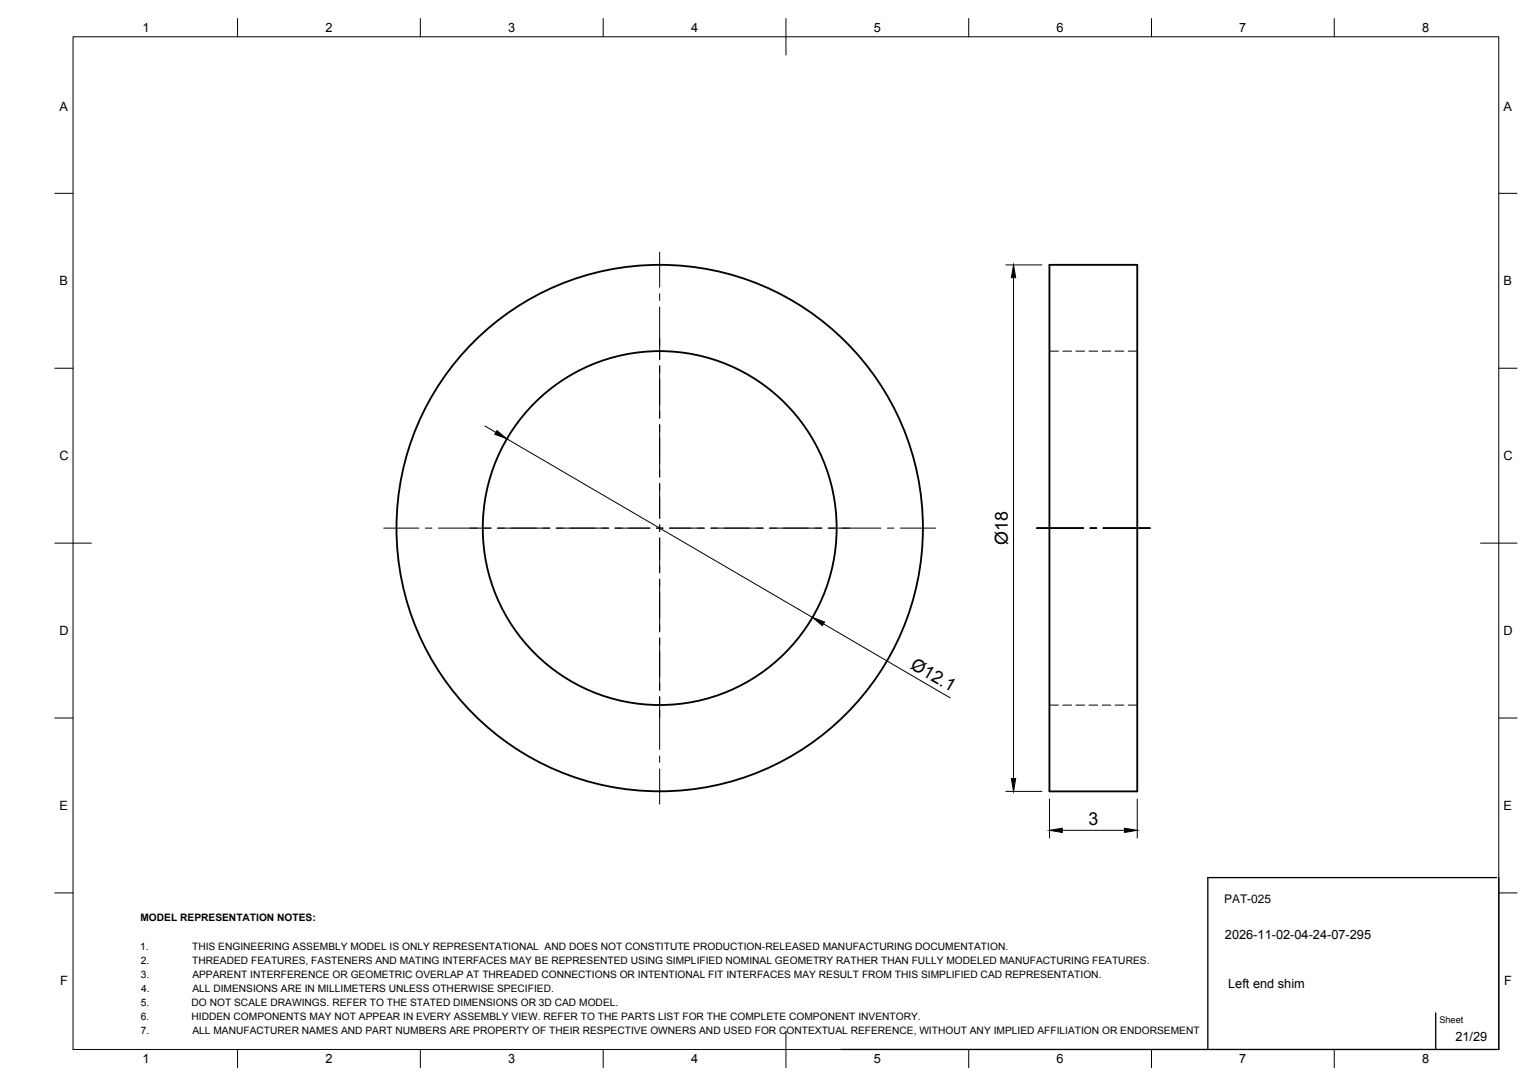
ISO-10303-21;
HEADER;
/* Generated by software containing ST-Developer
 * from STEP Tools, Inc. (www.steptools.com) 
 */

FILE_DESCRIPTION(
/* description */ ('Counter shaft with two pulleys and keyed hub'),
/* implementation_level */ '2;1');

FILE_NAME(
/* name */ 'Left end shim.step',
/* time_stamp */ '2026-10-27T10:46:10-07:00',
/* author */ (''),
/* organization */ (''),
/* preprocessor_version */ 'ST-DEVELOPER v20.2',
/* originating_system */ 'Autodesk Translation Framework v15.17.0.0',
/* authorisation */ '');

FILE_SCHEMA (('AUTOMOTIVE_DESIGN { 1 0 10303 214 3 1 1 }'));
ENDSEC;

DATA;
#10=MECHANICAL_DESIGN_GEOMETRIC_PRESENTATION_REPRESENTATION('',(#305),#10821);
#254=SHAPE_REPRESENTATION_RELATIONSHIP('SRR','None',#10942,#279);
#279=ADVANCED_BREP_SHAPE_REPRESENTATION('',(#330),#10810);
#305=STYLED_ITEM('',(#11128),#330);
#330=MANIFOLD_SOLID_BREP('Body1',#5589);
#399=FACE_BOUND('',#1097,.T.);
#400=FACE_BOUND('',#1099,.T.);
#519=PLANE('',#6139);
#520=PLANE('',#6140);
#721=FACE_OUTER_BOUND('',#1094,.T.);
#722=FACE_OUTER_BOUND('',#1095,.T.);
#723=FACE_OUTER_BOUND('',#1096,.T.);
#724=FACE_OUTER_BOUND('',#1098,.T.);
#1094=EDGE_LOOP('',(#4183,#4184,#4185,#4186));
#1095=EDGE_LOOP('',(#4187,#4188,#4189,#4190));
#1096=EDGE_LOOP('',(#4191));
#1097=EDGE_LOOP('',(#4192));
#1098=EDGE_LOOP('',(#4193));
#1099=EDGE_LOOP('',(#4194));
#1475=LINE('',#9363,#1864);
#1476=LINE('',#9369,#1865);
#1864=VECTOR('',#7243,0.605);
#1865=VECTOR('',#7250,0.9);
#2170=CIRCLE('',#6134,0.605);
#2171=CIRCLE('',#6135,0.605);
#2172=CIRCLE('',#6137,0.9);
#2173=CIRCLE('',#6138,0.9);
#2575=VERTEX_POINT('',#9360);
#2576=VERTEX_POINT('',#9362);
#2577=VERTEX_POINT('',#9366);
#2578=VERTEX_POINT('',#9368);
#3164=EDGE_CURVE('',#2575,#2575,#2170,.T.);
#3165=EDGE_CURVE('',#2575,#2576,#1475,.T.);
#3166=EDGE_CURVE('',#2576,#2576,#2171,.T.);
#3167=EDGE_CURVE('',#2577,#2577,#2172,.T.);
#3168=EDGE_CURVE('',#2577,#2578,#1476,.T.);
#3169=EDGE_CURVE('',#2578,#2578,#2173,.T.);
#4183=ORIENTED_EDGE('',*,*,#3164,.F.);
#4184=ORIENTED_EDGE('',*,*,#3165,.T.);
#4185=ORIENTED_EDGE('',*,*,#3166,.T.);
#4186=ORIENTED_EDGE('',*,*,#3165,.F.);
#4187=ORIENTED_EDGE('',*,*,#3167,.F.);
#4188=ORIENTED_EDGE('',*,*,#3168,.T.);
#4189=ORIENTED_EDGE('',*,*,#3169,.T.);
#4190=ORIENTED_EDGE('',*,*,#3168,.F.);
#4191=ORIENTED_EDGE('',*,*,#3167,.T.);
#4192=ORIENTED_EDGE('',*,*,#3164,.T.);
#4193=ORIENTED_EDGE('',*,*,#3169,.F.);
#4194=ORIENTED_EDGE('',*,*,#3166,.F.);
#5153=CYLINDRICAL_SURFACE('',#6133,0.605);
#5154=CYLINDRICAL_SURFACE('',#6136,0.9);
#5392=ADVANCED_FACE('',(#721),#5153,.F.);
#5393=ADVANCED_FACE('',(#722),#5154,.T.);
#5394=ADVANCED_FACE('',(#723,#399),#519,.T.);
#5395=ADVANCED_FACE('',(#724,#400),#520,.F.);
#5589=CLOSED_SHELL('',(#5392,#5393,#5394,#5395));
#6132=AXIS2_PLACEMENT_3D('',#9358,#7237,#7238);
#6133=AXIS2_PLACEMENT_3D('',#9359,#7239,#7240);
#6134=AXIS2_PLACEMENT_3D('',#9361,#7241,#7242);
#6135=AXIS2_PLACEMENT_3D('',#9364,#7244,#7245);
#6136=AXIS2_PLACEMENT_3D('',#9365,#7246,#7247);
#6137=AXIS2_PLACEMENT_3D('',#9367,#7248,#7249);
#6138=AXIS2_PLACEMENT_3D('',#9370,#7251,#7252);
#6139=AXIS2_PLACEMENT_3D('',#9371,#7253,#7254);
#6140=AXIS2_PLACEMENT_3D('',#9372,#7255,#7256);
#7237=DIRECTION('axis',(0.,0.,1.));
#7238=DIRECTION('refdir',(1.,0.,0.));
#7239=DIRECTION('center_axis',(0.,1.,0.));
#7240=DIRECTION('ref_axis',(1.,0.,0.));
#7241=DIRECTION('center_axis',(0.,-1.,0.));
#7242=DIRECTION('ref_axis',(1.,0.,0.));
#7243=DIRECTION('',(0.,-1.,0.));
#7244=DIRECTION('center_axis',(0.,-1.,0.));
#7245=DIRECTION('ref_axis',(1.,0.,0.));
#7246=DIRECTION('center_axis',(0.,1.,0.));
#7247=DIRECTION('ref_axis',(1.,0.,0.));
#7248=DIRECTION('center_axis',(0.,1.,0.));
#7249=DIRECTION('ref_axis',(1.,0.,0.));
#7250=DIRECTION('',(0.,-1.,0.));
#7251=DIRECTION('center_axis',(0.,1.,0.));
#7252=DIRECTION('ref_axis',(1.,0.,0.));
#7253=DIRECTION('center_axis',(0.,1.,0.));
#7254=DIRECTION('ref_axis',(1.,0.,0.));
#7255=DIRECTION('center_axis',(0.,1.,0.));
#7256=DIRECTION('ref_axis',(1.,0.,0.));
#9358=CARTESIAN_POINT('',(0.,0.,0.));
#9359=CARTESIAN_POINT('Origin',(0.,-5.5,4.53));
#9360=CARTESIAN_POINT('',(-0.605,-5.2,4.53));
#9361=CARTESIAN_POINT('Origin',(0.,-5.2,4.53));
#9362=CARTESIAN_POINT('',(-0.605,-5.5,4.53));
#9363=CARTESIAN_POINT('',(-0.605,-5.5,4.53));
#9364=CARTESIAN_POINT('Origin',(0.,-5.5,4.53));
#9365=CARTESIAN_POINT('Origin',(0.,-5.5,4.53));
#9366=CARTESIAN_POINT('',(-0.9,-5.2,4.53));
#9367=CARTESIAN_POINT('Origin',(0.,-5.2,4.53));
#9368=CARTESIAN_POINT('',(-0.9,-5.5,4.53));
#9369=CARTESIAN_POINT('',(-0.9,-5.5,4.53));
#9370=CARTESIAN_POINT('Origin',(0.,-5.5,4.53));
#9371=CARTESIAN_POINT('Origin',(0.,-5.2,4.53));
#9372=CARTESIAN_POINT('Origin',(0.,-5.5,4.53));
#10780=UNCERTAINTY_MEASURE_WITH_UNIT(LENGTH_MEASURE(0.001),#10822,
'DISTANCE_ACCURACY_VALUE',
'Maximum model space distance between geometric entities at asserted c
onnectivities');
#10791=UNCERTAINTY_MEASURE_WITH_UNIT(LENGTH_MEASURE(0.001),#10822,
'DISTANCE_ACCURACY_VALUE',
'Maximum model space distance between geometric entities at asserted c
onnectivities');
#10810=(
GEOMETRIC_REPRESENTATION_CONTEXT(3)
GLOBAL_UNCERTAINTY_ASSIGNED_CONTEXT((#10780))
GLOBAL_UNIT_ASSIGNED_CONTEXT((#10822,#10824,#10825))
REPRESENTATION_CONTEXT('','3D')
);
#10821=(
GEOMETRIC_REPRESENTATION_CONTEXT(3)
GLOBAL_UNCERTAINTY_ASSIGNED_CONTEXT((#10791))
GLOBAL_UNIT_ASSIGNED_CONTEXT((#10822,#10824,#10825))
REPRESENTATION_CONTEXT('','3D')
);
#10822=(
LENGTH_UNIT()
NAMED_UNIT(*)
SI_UNIT(.CENTI.,.METRE.)
);
#10824=(
NAMED_UNIT(*)
PLANE_ANGLE_UNIT()
SI_UNIT($,.RADIAN.)
);
#10825=(
NAMED_UNIT(*)
SI_UNIT($,.STERADIAN.)
SOLID_ANGLE_UNIT()
);
#10844=SHAPE_DEFINITION_REPRESENTATION(#10892,#10942);
#10892=PRODUCT_DEFINITION_SHAPE('',$,#10972);
#10942=SHAPE_REPRESENTATION('',(#6132),#10810);
#10953=PRODUCT_DEFINITION_CONTEXT('part definition',#11042,'design');
#10972=PRODUCT_DEFINITION('Left end shim','Left end shim',#11001,#10953);
#11001=PRODUCT_DEFINITION_FORMATION('',$,#11062);
#11042=APPLICATION_CONTEXT(
'Core Data for Automotive Mechanical Design Process');
#11043=PRODUCT_CONTEXT('part definition',#11042,'mechanical');
#11062=PRODUCT('Left end shim','Left end shim','Left end shim',(#11043));
#11122=COLOUR_RGB('Sky Blue',0.24,0.69,0.87);
#11123=FILL_AREA_STYLE_COLOUR('',#11122);
#11124=FILL_AREA_STYLE('',(#11123));
#11125=SURFACE_STYLE_FILL_AREA(#11124);
#11126=SURFACE_SIDE_STYLE('',(#11125));
#11127=SURFACE_STYLE_USAGE(.BOTH.,#11126);
#11128=PRESENTATION_STYLE_ASSIGNMENT((#11127));
ENDSEC;
END-ISO-10303-21;
